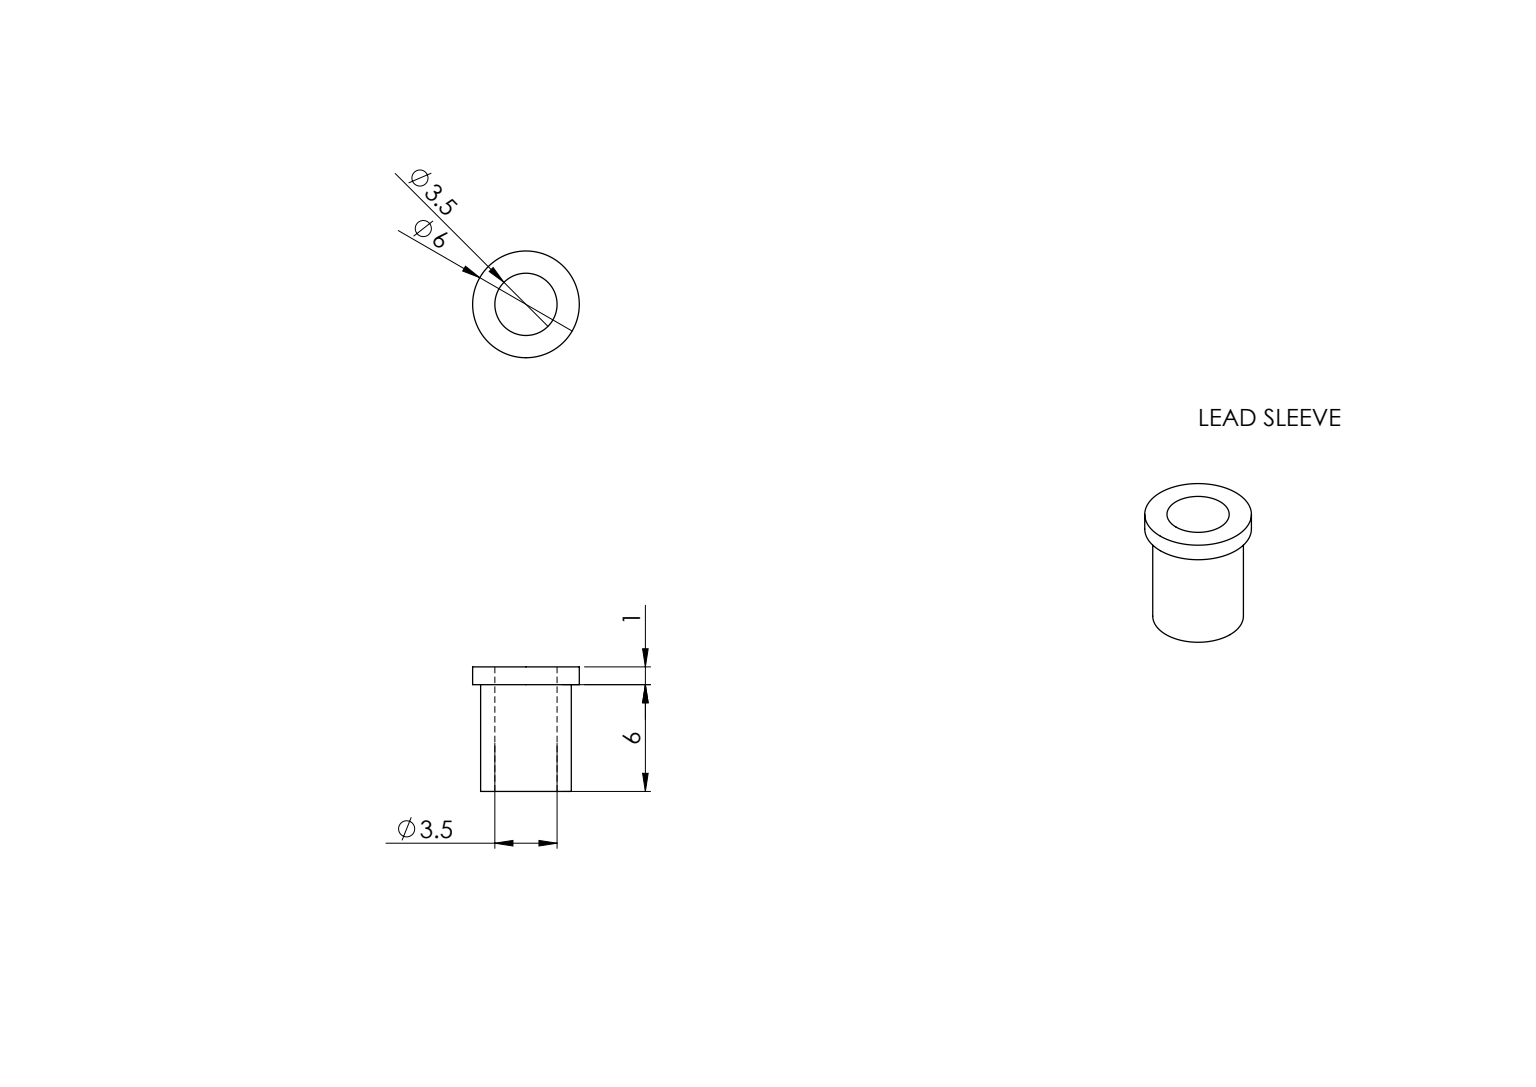
ISO-10303-21;
HEADER;
FILE_DESCRIPTION (('STEP AP214'),
    '1' );
FILE_NAME ('lead sleeve.step',
    '2026-10-27T10:49:47',
    ( '' ),
    ( '' ),
    'SwSTEP 2.0',
    'SolidWorks 2026',
    '' );
FILE_SCHEMA (( 'AUTOMOTIVE_DESIGN' ));
ENDSEC;

DATA;
#24=CARTESIAN_POINT ( 'NONE',  ( 0.000000000000000000, -53.00000000000000000, 0.000000000000000000 ) ) ;
#28=PRODUCT_DEFINITION_SHAPE ( 'NONE', 'NONE',  #6653 ) ;
#101=DIRECTION ( 'NONE',  ( 0.000000000000000000, 1.000000000000000000, 0.000000000000000000 ) ) ;
#135=ORIENTED_EDGE ( 'NONE', *, *, #4743, .T. ) ;
#208=ORIENTED_EDGE ( 'NONE', *, *, #3669, .T. ) ;
#212=EDGE_LOOP ( 'NONE', ( #4167, #4581 ) ) ;
#286=DIRECTION ( 'NONE',  ( -0.000000000000000000, 1.000000000000000000, -0.000000000000000000 ) ) ;
#296=VERTEX_POINT ( 'NONE', #8506 ) ;
#306=PRODUCT_DEFINITION_CONTEXT ( 'detailed design', #4038, 'design' ) ;
#328=CARTESIAN_POINT ( 'NONE',  ( 0.000000000000000000, -47.00000000000000000, 0.000000000000000000 ) ) ;
#391=EDGE_CURVE ( 'NONE', #8882, #738, #2591, .T. ) ;
#423=ORIENTED_EDGE ( 'NONE', *, *, #8631, .F. ) ;
#456=( NAMED_UNIT ( * ) SI_UNIT ( $, .STERADIAN. ) SOLID_ANGLE_UNIT ( ) );
#464=DIRECTION ( 'NONE',  ( -0.000000000000000000, -1.000000000000000000, -0.000000000000000000 ) ) ;
#468=ORIENTED_EDGE ( 'NONE', *, *, #7764, .T. ) ;
#469=CARTESIAN_POINT ( 'NONE',  ( 2.143131898507868051E-16, -53.00000000000000000, -1.749999999999999778 ) ) ;
#515=FACE_OUTER_BOUND ( 'NONE', #8742, .T. ) ;
#552=LINE ( 'NONE', #1253, #8953 ) ;
#596=CARTESIAN_POINT ( 'NONE',  ( 0.000000000000000000, -53.00000000000000000, 0.000000000000000000 ) ) ;
#631=ORIENTED_EDGE ( 'NONE', *, *, #8631, .T. ) ;
#673=ORIENTED_EDGE ( 'NONE', *, *, #5568, .T. ) ;
#711=CYLINDRICAL_SURFACE ( 'NONE', #5192, 1.749999999999999778 ) ;
#738=VERTEX_POINT ( 'NONE', #4144 ) ;
#791=VERTEX_POINT ( 'NONE', #4553 ) ;
#888=AXIS2_PLACEMENT_3D ( 'NONE', #4026, #9081, #6861 ) ;
#903=DIRECTION ( 'NONE',  ( 1.000000000000000000, 0.000000000000000000, 0.000000000000000000 ) ) ;
#945=AXIS2_PLACEMENT_3D ( 'NONE', #2361, #8822, #2458 ) ;
#968=ORIENTED_EDGE ( 'NONE', *, *, #8122, .T. ) ;
#1000=EDGE_CURVE ( 'NONE', #4607, #791, #3032, .T. ) ;
#1019=ORIENTED_EDGE ( 'NONE', *, *, #3908, .F. ) ;
#1038=VECTOR ( 'NONE', #2949, 1000.000000000000000 ) ;
#1070=CARTESIAN_POINT ( 'NONE',  ( 0.000000000000000000, -47.00000000000000000, 2.549999999999999822 ) ) ;
#1077=EDGE_CURVE ( 'NONE', #791, #6502, #552, .T. ) ;
#1085=DIRECTION ( 'NONE',  ( 0.000000000000000000, -1.000000000000000000, 0.000000000000000000 ) ) ;
#1134=CARTESIAN_POINT ( 'NONE',  ( 0.000000000000000000, -47.00000000000000000, 0.000000000000000000 ) ) ;
#1140=CARTESIAN_POINT ( 'NONE',  ( 0.000000000000000000, -47.00000000000000000, -2.999999999999999556 ) ) ;
#1143=LINE ( 'NONE', #6765, #5493 ) ;
#1210=SHAPE_DEFINITION_REPRESENTATION ( #28, #2490 ) ;
#1249=EDGE_CURVE ( 'NONE', #1724, #4568, #3611, .T. ) ;
#1253=CARTESIAN_POINT ( 'NONE',  ( 0.000000000000000000, -46.00000000000000000, -2.999999999999999556 ) ) ;
#1337=CARTESIAN_POINT ( 'NONE',  ( 0.000000000000000000, -53.00000000000000000, 0.000000000000000000 ) ) ;
#1386=ADVANCED_FACE ( 'NONE', ( #5610 ), #2170, .F. ) ;
#1441=DIRECTION ( 'NONE',  ( 0.000000000000000000, 0.000000000000000000, 1.000000000000000000 ) ) ;
#1472=DIRECTION ( 'NONE',  ( 0.000000000000000000, 1.000000000000000000, 0.000000000000000000 ) ) ;
#1490=DIRECTION ( 'NONE',  ( 0.000000000000000000, 1.000000000000000000, 0.000000000000000000 ) ) ;
#1516=UNCERTAINTY_MEASURE_WITH_UNIT (LENGTH_MEASURE( 1.000000000000000082E-05 ), #2714, 'distance_accuracy_value', 'NONE');
#1641=DIRECTION ( 'NONE',  ( 0.000000000000000000, 0.000000000000000000, 1.000000000000000000 ) ) ;
#1689=CARTESIAN_POINT ( 'NONE',  ( 0.000000000000000000, -53.00000000000000000, 2.549999999999999822 ) ) ;
#1724=VERTEX_POINT ( 'NONE', #8575 ) ;
#1835=CARTESIAN_POINT ( 'NONE',  ( 3.122849337825750419E-16, -53.00000000000000000, -2.549999999999999822 ) ) ;
#1844=VERTEX_POINT ( 'NONE', #469 ) ;
#1957=CARTESIAN_POINT ( 'NONE',  ( 0.000000000000000000, -53.00000000000000000, 0.000000000000000000 ) ) ;
#1993=DIRECTION ( 'NONE',  ( 0.000000000000000000, -1.000000000000000000, 0.000000000000000000 ) ) ;
#2043=DIRECTION ( 'NONE',  ( 0.000000000000000000, 0.000000000000000000, 1.000000000000000000 ) ) ;
#2148=MANIFOLD_SOLID_BREP ( 'Boss-Extrude1', #7133 ) ;
#2160=ORIENTED_EDGE ( 'NONE', *, *, #6275, .F. ) ;
#2170=CYLINDRICAL_SURFACE ( 'NONE', #2847, 1.749999999999999778 ) ;
#2214=DIRECTION ( 'NONE',  ( 1.000000000000000000, 0.000000000000000000, 0.000000000000000000 ) ) ;
#2216=AXIS2_PLACEMENT_3D ( 'NONE', #3437, #6390, #7094 ) ;
#2281=ORIENTED_EDGE ( 'NONE', *, *, #1000, .T. ) ;
#2361=CARTESIAN_POINT ( 'NONE',  ( 0.000000000000000000, -46.00000000000000000, 0.000000000000000000 ) ) ;
#2441=AXIS2_PLACEMENT_3D ( 'NONE', #5660, #7852, #2043 ) ;
#2458=DIRECTION ( 'NONE',  ( 0.000000000000000000, -0.000000000000000000, 1.000000000000000000 ) ) ;
#2464=DIRECTION ( 'NONE',  ( 0.000000000000000000, 0.000000000000000000, 1.000000000000000000 ) ) ;
#2479=FACE_BOUND ( 'NONE', #8500, .T. ) ;
#2490=SHAPE_REPRESENTATION ( 'lead sleeve', ( #888 ), #5908 ) ;
#2499=STYLED_ITEM ( 'NONE', ( #8555 ), #6298 ) ;
#2531=CARTESIAN_POINT ( 'NONE',  ( 0.000000000000000000, -53.00000000000000000, 0.000000000000000000 ) ) ;
#2560=DIRECTION ( 'NONE',  ( 0.000000000000000000, 1.000000000000000000, 0.000000000000000000 ) ) ;
#2583=DIRECTION ( 'NONE',  ( 0.000000000000000000, -1.000000000000000000, 0.000000000000000000 ) ) ;
#2591=CIRCLE ( 'NONE', #5546, 1.750000000000000222 ) ;
#2685=AXIS2_PLACEMENT_3D ( 'NONE', #8707, #101, #1641 ) ;
#2705=CARTESIAN_POINT ( 'NONE',  ( 0.000000000000000000, -46.00000000000000000, 0.000000000000000000 ) ) ;
#2714=( LENGTH_UNIT ( ) NAMED_UNIT ( * ) SI_UNIT ( .MILLI., .METRE. ) );
#2733=APPLICATION_CONTEXT ( 'automotive_design' ) ;
#2790=CARTESIAN_POINT ( 'NONE',  ( 0.000000000000000000, -53.00000000000000000, 0.000000000000000000 ) ) ;
#2804=( NAMED_UNIT ( * ) PLANE_ANGLE_UNIT ( ) SI_UNIT ( $, .RADIAN. ) );
#2806=ORIENTED_EDGE ( 'NONE', *, *, #8722, .T. ) ;
#2847=AXIS2_PLACEMENT_3D ( 'NONE', #596, #5567, #4991 ) ;
#2852=SURFACE_SIDE_STYLE ('',( #6497 ) ) ;
#2877=ADVANCED_FACE ( 'NONE', ( #7837 ), #711, .F. ) ;
#2921=LINE ( 'NONE', #5738, #5025 ) ;
#2949=DIRECTION ( 'NONE',  ( -0.000000000000000000, -1.000000000000000000, -0.000000000000000000 ) ) ;
#2991=ORIENTED_EDGE ( 'NONE', *, *, #5699, .F. ) ;
#3032=CIRCLE ( 'NONE', #7773, 2.999999999999999556 ) ;
#3139=AXIS2_PLACEMENT_3D ( 'NONE', #2790, #7100, #4360 ) ;
#3140=ORIENTED_EDGE ( 'NONE', *, *, #7764, .F. ) ;
#3143=FACE_OUTER_BOUND ( 'NONE', #5079, .T. ) ;
#3160=FACE_OUTER_BOUND ( 'NONE', #9177, .T. ) ;
#3183=ORIENTED_EDGE ( 'NONE', *, *, #8443, .F. ) ;
#3297=MECHANICAL_DESIGN_GEOMETRIC_PRESENTATION_REPRESENTATION('',(#8174),#4159);
#3303=FACE_OUTER_BOUND ( 'NONE', #6297, .T. ) ;
#3309=DIRECTION ( 'NONE',  ( 0.000000000000000000, 0.000000000000000000, 1.000000000000000000 ) ) ;
#3437=CARTESIAN_POINT ( 'NONE',  ( 0.000000000000000000, -46.00000000000000000, 0.000000000000000000 ) ) ;
#3447=CARTESIAN_POINT ( 'NONE',  ( 0.000000000000000000, -47.00000000000000000, 0.000000000000000000 ) ) ;
#3471=AXIS2_PLACEMENT_3D ( 'NONE', #1337, #7896, #2214 ) ;
#3502=LINE ( 'NONE', #7825, #9116 ) ;
#3515=DIRECTION ( 'NONE',  ( 0.000000000000000000, 0.000000000000000000, 1.000000000000000000 ) ) ;
#3538=( NAMED_UNIT ( * ) SI_UNIT ( $, .STERADIAN. ) SOLID_ANGLE_UNIT ( ) );
#3561=ORIENTED_EDGE ( 'NONE', *, *, #1000, .F. ) ;
#3611=CIRCLE ( 'NONE', #3471, 2.549999999999999822 ) ;
#3663=PLANE ( 'NONE',  #945 ) ;
#3669=EDGE_CURVE ( 'NONE', #6874, #296, #8611, .T. ) ;
#3767=AXIS2_PLACEMENT_3D ( 'NONE', #5405, #1490, #1441 ) ;
#3796=ADVANCED_FACE ( 'NONE', ( #7193 ), #4992, .T. ) ;
#3845=ORIENTED_EDGE ( 'NONE', *, *, #6275, .T. ) ;
#3896=ORIENTED_EDGE ( 'NONE', *, *, #1249, .F. ) ;
#3908=EDGE_CURVE ( 'NONE', #4607, #5775, #4385, .T. ) ;
#3986=DIRECTION ( 'NONE',  ( -0.000000000000000000, 1.000000000000000000, -0.000000000000000000 ) ) ;
#3997=( LENGTH_UNIT ( ) NAMED_UNIT ( * ) SI_UNIT ( .MILLI., .METRE. ) );
#4026=CARTESIAN_POINT ( 'NONE',  ( 0.000000000000000000, 0.000000000000000000, 0.000000000000000000 ) ) ;
#4038=APPLICATION_CONTEXT ( 'automotive_design' ) ;
#4048=CYLINDRICAL_SURFACE ( 'NONE', #6897, 2.549999999999999822 ) ;
#4111=CARTESIAN_POINT ( 'NONE',  ( 0.000000000000000000, -53.00000000000000000, 1.749999999999999778 ) ) ;
#4144=CARTESIAN_POINT ( 'NONE',  ( 2.143131898507868544E-16, -46.00000000000000000, -1.750000000000000222 ) ) ;
#4159=( GEOMETRIC_REPRESENTATION_CONTEXT ( 3 ) GLOBAL_UNCERTAINTY_ASSIGNED_CONTEXT ( ( #7422 ) ) GLOBAL_UNIT_ASSIGNED_CONTEXT ( ( #3997, #6778, #456 ) ) REPRESENTATION_CONTEXT ( 'NONE', 'WORKASPACE' ) );
#4167=ORIENTED_EDGE ( 'NONE', *, *, #391, .F. ) ;
#4175=FACE_OUTER_BOUND ( 'NONE', #8554, .T. ) ;
#4279=MECHANICAL_DESIGN_GEOMETRIC_PRESENTATION_REPRESENTATION('',(#2499),#6348);
#4360=DIRECTION ( 'NONE',  ( 0.000000000000000000, 0.000000000000000000, 1.000000000000000000 ) ) ;
#4385=LINE ( 'NONE', #7215, #1038 ) ;
#4400=ORIENTED_EDGE ( 'NONE', *, *, #5699, .T. ) ;
#4475=DIRECTION ( 'NONE',  ( 0.000000000000000000, -0.000000000000000000, 1.000000000000000000 ) ) ;
#4553=CARTESIAN_POINT ( 'NONE',  ( 0.000000000000000000, -46.00000000000000000, -2.999999999999999556 ) ) ;
#4568=VERTEX_POINT ( 'NONE', #1835 ) ;
#4581=ORIENTED_EDGE ( 'NONE', *, *, #6056, .F. ) ;
#4607=VERTEX_POINT ( 'NONE', #6052 ) ;
#4638=ORIENTED_EDGE ( 'NONE', *, *, #1077, .T. ) ;
#4643=CARTESIAN_POINT ( 'NONE',  ( 0.000000000000000000, -46.00000000000000000, 0.000000000000000000 ) ) ;
#4660=EDGE_LOOP ( 'NONE', ( #4753, #4816 ) ) ;
#4666=PLANE ( 'NONE',  #5776 ) ;
#4687=CARTESIAN_POINT ( 'NONE',  ( 0.000000000000000000, -53.00000000000000000, 0.000000000000000000 ) ) ;
#4690=CARTESIAN_POINT ( 'NONE',  ( 0.000000000000000000, -47.00000000000000000, 0.000000000000000000 ) ) ;
#4696=DIRECTION ( 'NONE',  ( 0.000000000000000000, 0.000000000000000000, -1.000000000000000000 ) ) ;
#4743=EDGE_CURVE ( 'NONE', #296, #6874, #7917, .T. ) ;
#4746=AXIS2_PLACEMENT_3D ( 'NONE', #4687, #6027, #8864 ) ;
#4750=ORIENTED_EDGE ( 'NONE', *, *, #4743, .F. ) ;
#4753=ORIENTED_EDGE ( 'NONE', *, *, #7099, .F. ) ;
#4783=CARTESIAN_POINT ( 'NONE',  ( 0.000000000000000000, -53.00000000000000000, 0.000000000000000000 ) ) ;
#4788=DIRECTION ( 'NONE',  ( 0.000000000000000000, 1.000000000000000000, 0.000000000000000000 ) ) ;
#4816=ORIENTED_EDGE ( 'NONE', *, *, #5422, .F. ) ;
#4825=DIRECTION ( 'NONE',  ( 1.000000000000000000, 0.000000000000000000, 0.000000000000000000 ) ) ;
#4906=EDGE_LOOP ( 'NONE', ( #468, #968, #8047, #3183 ) ) ;
#4921=PRODUCT ( 'lead sleeve', 'lead sleeve', '', ( #7531 ) ) ;
#4991=DIRECTION ( 'NONE',  ( 0.000000000000000000, 0.000000000000000000, 1.000000000000000000 ) ) ;
#4992=CYLINDRICAL_SURFACE ( 'NONE', #3139, 2.549999999999999822 ) ;
#4998=PRODUCT_DEFINITION_FORMATION_WITH_SPECIFIED_SOURCE ( 'ANY', '', #4921, .NOT_KNOWN. ) ;
#5025=VECTOR ( 'NONE', #7755, 1000.000000000000000 ) ;
#5079=EDGE_LOOP ( 'NONE', ( #5622, #3845 ) ) ;
#5160=ORIENTED_EDGE ( 'NONE', *, *, #8722, .F. ) ;
#5192=AXIS2_PLACEMENT_3D ( 'NONE', #7003, #8445, #3515 ) ;
#5303=EDGE_LOOP ( 'NONE', ( #2160, #673, #135, #5160 ) ) ;
#5355=DIRECTION ( 'NONE',  ( 0.000000000000000000, -0.000000000000000000, -1.000000000000000000 ) ) ;
#5384=VERTEX_POINT ( 'NONE', #4111 ) ;
#5405=CARTESIAN_POINT ( 'NONE',  ( 0.000000000000000000, -47.00000000000000000, 0.000000000000000000 ) ) ;
#5422=EDGE_CURVE ( 'NONE', #5775, #6502, #7482, .T. ) ;
#5429=DIRECTION ( 'NONE',  ( 0.000000000000000000, -1.000000000000000000, 0.000000000000000000 ) ) ;
#5470=ORIENTED_EDGE ( 'NONE', *, *, #8443, .T. ) ;
#5493=VECTOR ( 'NONE', #3986, 1000.000000000000000 ) ;
#5546=AXIS2_PLACEMENT_3D ( 'NONE', #7287, #1472, #6443 ) ;
#5553=AXIS2_PLACEMENT_3D ( 'NONE', #1957, #6929, #6183 ) ;
#5567=DIRECTION ( 'NONE',  ( -0.000000000000000000, 1.000000000000000000, -0.000000000000000000 ) ) ;
#5568=EDGE_CURVE ( 'NONE', #4568, #296, #3502, .T. ) ;
#5610=FACE_OUTER_BOUND ( 'NONE', #4906, .T. ) ;
#5622=ORIENTED_EDGE ( 'NONE', *, *, #1249, .T. ) ;
#5660=CARTESIAN_POINT ( 'NONE',  ( 0.000000000000000000, -46.00000000000000000, 0.000000000000000000 ) ) ;
#5669=SHAPE_REPRESENTATION_RELATIONSHIP ( 'NONE' , 'NONE' ,  #2490, #6298 ) ;
#5699=EDGE_CURVE ( 'NONE', #1844, #5384, #8960, .T. ) ;
#5704=ADVANCED_FACE ( 'NONE', ( #3303 ), #4048, .T. ) ;
#5712=SURFACE_STYLE_USAGE ( .BOTH. , #2852 ) ;
#5738=CARTESIAN_POINT ( 'NONE',  ( 2.143131898507868051E-16, -53.00000000000000000, -1.749999999999999778 ) ) ;
#5775=VERTEX_POINT ( 'NONE', #8964 ) ;
#5776=AXIS2_PLACEMENT_3D ( 'NONE', #2531, #1085, #5355 ) ;
#5807=CARTESIAN_POINT ( 'NONE',  ( 0.000000000000000000, -46.00000000000000000, 1.750000000000000222 ) ) ;
#5808=ORIENTED_EDGE ( 'NONE', *, *, #8122, .F. ) ;
#5864=PLANE ( 'NONE',  #6294 ) ;
#5872=ADVANCED_FACE ( 'NONE', ( #2479, #8104 ), #5864, .F. ) ;
#5908=( GEOMETRIC_REPRESENTATION_CONTEXT ( 3 ) GLOBAL_UNCERTAINTY_ASSIGNED_CONTEXT ( ( #1516 ) ) GLOBAL_UNIT_ASSIGNED_CONTEXT ( ( #2714, #6098, #6983 ) ) REPRESENTATION_CONTEXT ( 'NONE', 'WORKASPACE' ) );
#5980=FACE_BOUND ( 'NONE', #212, .T. ) ;
#5994=CIRCLE ( 'NONE', #7783, 2.549999999999999822 ) ;
#6024=ORIENTED_EDGE ( 'NONE', *, *, #391, .T. ) ;
#6027=DIRECTION ( 'NONE',  ( 0.000000000000000000, -1.000000000000000000, 0.000000000000000000 ) ) ;
#6052=CARTESIAN_POINT ( 'NONE',  ( 3.673940397442059375E-16, -46.00000000000000000, 2.999999999999999556 ) ) ;
#6056=EDGE_CURVE ( 'NONE', #738, #8882, #6431, .T. ) ;
#6076=DIRECTION ( 'NONE',  ( -0.000000000000000000, -1.000000000000000000, -0.000000000000000000 ) ) ;
#6098=( NAMED_UNIT ( * ) PLANE_ANGLE_UNIT ( ) SI_UNIT ( $, .RADIAN. ) );
#6119=ORIENTED_EDGE ( 'NONE', *, *, #5422, .T. ) ;
#6139=CYLINDRICAL_SURFACE ( 'NONE', #6819, 2.999999999999999556 ) ;
#6174=ADVANCED_FACE ( 'NONE', ( #3160, #5980 ), #3663, .T. ) ;
#6183=DIRECTION ( 'NONE',  ( 0.000000000000000000, 0.000000000000000000, -1.000000000000000000 ) ) ;
#6275=EDGE_CURVE ( 'NONE', #4568, #1724, #5994, .T. ) ;
#6294=AXIS2_PLACEMENT_3D ( 'NONE', #328, #8704, #4475 ) ;
#6297=EDGE_LOOP ( 'NONE', ( #6732, #3896, #2806, #208 ) ) ;
#6298=ADVANCED_BREP_SHAPE_REPRESENTATION ( '', ( #2148, #888 ), #5908 ) ;
#6348=( GEOMETRIC_REPRESENTATION_CONTEXT ( 3 ) GLOBAL_UNCERTAINTY_ASSIGNED_CONTEXT ( ( #6534 ) ) GLOBAL_UNIT_ASSIGNED_CONTEXT ( ( #7068, #2804, #3538 ) ) REPRESENTATION_CONTEXT ( 'NONE', 'WORKASPACE' ) );
#6390=DIRECTION ( 'NONE',  ( -0.000000000000000000, -1.000000000000000000, -0.000000000000000000 ) ) ;
#6431=CIRCLE ( 'NONE', #2441, 1.750000000000000222 ) ;
#6443=DIRECTION ( 'NONE',  ( 0.000000000000000000, 0.000000000000000000, 1.000000000000000000 ) ) ;
#6497=SURFACE_STYLE_FILL_AREA ( #7728 ) ;
#6502=VERTEX_POINT ( 'NONE', #1140 ) ;
#6534=UNCERTAINTY_MEASURE_WITH_UNIT (LENGTH_MEASURE( 1.000000000000000082E-05 ), #7068, 'distance_accuracy_value', 'NONE');
#6653=PRODUCT_DEFINITION ( 'UNKNOWN', '', #4998, #306 ) ;
#6732=ORIENTED_EDGE ( 'NONE', *, *, #5568, .F. ) ;
#6765=CARTESIAN_POINT ( 'NONE',  ( 0.000000000000000000, -53.00000000000000000, 1.749999999999999778 ) ) ;
#6778=( NAMED_UNIT ( * ) PLANE_ANGLE_UNIT ( ) SI_UNIT ( $, .RADIAN. ) );
#6819=AXIS2_PLACEMENT_3D ( 'NONE', #2705, #464, #4696 ) ;
#6861=DIRECTION ( 'NONE',  ( 1.000000000000000000, 0.000000000000000000, 0.000000000000000000 ) ) ;
#6874=VERTEX_POINT ( 'NONE', #1070 ) ;
#6897=AXIS2_PLACEMENT_3D ( 'NONE', #4783, #8186, #2464 ) ;
#6929=DIRECTION ( 'NONE',  ( 0.000000000000000000, -1.000000000000000000, 0.000000000000000000 ) ) ;
#6983=( NAMED_UNIT ( * ) SI_UNIT ( $, .STERADIAN. ) SOLID_ANGLE_UNIT ( ) );
#7003=CARTESIAN_POINT ( 'NONE',  ( 0.000000000000000000, -53.00000000000000000, 0.000000000000000000 ) ) ;
#7068=( LENGTH_UNIT ( ) NAMED_UNIT ( * ) SI_UNIT ( .MILLI., .METRE. ) );
#7094=DIRECTION ( 'NONE',  ( 0.000000000000000000, 0.000000000000000000, -1.000000000000000000 ) ) ;
#7096=ADVANCED_FACE ( 'NONE', ( #515 ), #6139, .T. ) ;
#7099=EDGE_CURVE ( 'NONE', #6502, #5775, #7566, .T. ) ;
#7100=DIRECTION ( 'NONE',  ( -0.000000000000000000, 1.000000000000000000, -0.000000000000000000 ) ) ;
#7115=CIRCLE ( 'NONE', #4746, 1.749999999999999778 ) ;
#7133=CLOSED_SHELL ( 'NONE', ( #7096, #1386, #3796, #8797, #5704, #2877, #6174, #5872, #7979 ) ) ;
#7161=EDGE_LOOP ( 'NONE', ( #3140, #2991 ) ) ;
#7193=FACE_OUTER_BOUND ( 'NONE', #5303, .T. ) ;
#7215=CARTESIAN_POINT ( 'NONE',  ( 3.673940397442059375E-16, -46.00000000000000000, 2.999999999999999556 ) ) ;
#7282=AXIS2_PLACEMENT_3D ( 'NONE', #4690, #5429, #4825 ) ;
#7287=CARTESIAN_POINT ( 'NONE',  ( 0.000000000000000000, -46.00000000000000000, 0.000000000000000000 ) ) ;
#7299=ORIENTED_EDGE ( 'NONE', *, *, #7099, .T. ) ;
#7392=COLOUR_RGB ( '',0.8941176470588234615, 0.8941176470588234615, 0.8941176470588234615 ) ;
#7422=UNCERTAINTY_MEASURE_WITH_UNIT (LENGTH_MEASURE( 1.000000000000000082E-05 ), #3997, 'distance_accuracy_value', 'NONE');
#7482=CIRCLE ( 'NONE', #3767, 2.999999999999999556 ) ;
#7484=DIRECTION ( 'NONE',  ( 0.000000000000000000, 0.000000000000000000, 1.000000000000000000 ) ) ;
#7530=ORIENTED_EDGE ( 'NONE', *, *, #3908, .T. ) ;
#7531=PRODUCT_CONTEXT ( 'NONE', #2733, 'mechanical' ) ;
#7544=ORIENTED_EDGE ( 'NONE', *, *, #3669, .F. ) ;
#7566=CIRCLE ( 'NONE', #8747, 2.999999999999999556 ) ;
#7728=FILL_AREA_STYLE ('',( #8473 ) ) ;
#7755=DIRECTION ( 'NONE',  ( -0.000000000000000000, 1.000000000000000000, -0.000000000000000000 ) ) ;
#7764=EDGE_CURVE ( 'NONE', #5384, #1844, #7115, .T. ) ;
#7773=AXIS2_PLACEMENT_3D ( 'NONE', #4643, #2560, #7484 ) ;
#7780=DIRECTION ( 'NONE',  ( -0.000000000000000000, 1.000000000000000000, -0.000000000000000000 ) ) ;
#7783=AXIS2_PLACEMENT_3D ( 'NONE', #24, #1993, #903 ) ;
#7825=CARTESIAN_POINT ( 'NONE',  ( 3.122849337825750419E-16, -53.00000000000000000, -2.549999999999999822 ) ) ;
#7837=FACE_OUTER_BOUND ( 'NONE', #8770, .T. ) ;
#7852=DIRECTION ( 'NONE',  ( 0.000000000000000000, 1.000000000000000000, 0.000000000000000000 ) ) ;
#7892=CYLINDRICAL_SURFACE ( 'NONE', #2216, 2.999999999999999556 ) ;
#7896=DIRECTION ( 'NONE',  ( 0.000000000000000000, -1.000000000000000000, 0.000000000000000000 ) ) ;
#7917=CIRCLE ( 'NONE', #8064, 2.549999999999999822 ) ;
#7921=LINE ( 'NONE', #1689, #8761 ) ;
#7979=ADVANCED_FACE ( 'NONE', ( #4175 ), #7892, .T. ) ;
#8047=ORIENTED_EDGE ( 'NONE', *, *, #6056, .T. ) ;
#8064=AXIS2_PLACEMENT_3D ( 'NONE', #1134, #2583, #8847 ) ;
#8104=FACE_OUTER_BOUND ( 'NONE', #4660, .T. ) ;
#8108=FACE_BOUND ( 'NONE', #7161, .T. ) ;
#8122=EDGE_CURVE ( 'NONE', #1844, #738, #2921, .T. ) ;
#8174=STYLED_ITEM('',(#9239),#2148);
#8186=DIRECTION ( 'NONE',  ( -0.000000000000000000, 1.000000000000000000, -0.000000000000000000 ) ) ;
#8323=CIRCLE ( 'NONE', #2685, 2.999999999999999556 ) ;
#8443=EDGE_CURVE ( 'NONE', #5384, #8882, #1143, .T. ) ;
#8445=DIRECTION ( 'NONE',  ( -0.000000000000000000, 1.000000000000000000, -0.000000000000000000 ) ) ;
#8473=FILL_AREA_STYLE_COLOUR ( '', #7392 ) ;
#8500=EDGE_LOOP ( 'NONE', ( #7544, #4750 ) ) ;
#8506=CARTESIAN_POINT ( 'NONE',  ( 3.122849337825750419E-16, -47.00000000000000000, -2.549999999999999822 ) ) ;
#8554=EDGE_LOOP ( 'NONE', ( #1019, #423, #4638, #7299 ) ) ;
#8555=PRESENTATION_STYLE_ASSIGNMENT (( #5712 ) ) ;
#8575=CARTESIAN_POINT ( 'NONE',  ( 0.000000000000000000, -53.00000000000000000, 2.549999999999999822 ) ) ;
#8611=CIRCLE ( 'NONE', #7282, 2.549999999999999822 ) ;
#8631=EDGE_CURVE ( 'NONE', #791, #4607, #8323, .T. ) ;
#8704=DIRECTION ( 'NONE',  ( 0.000000000000000000, 1.000000000000000000, 0.000000000000000000 ) ) ;
#8707=CARTESIAN_POINT ( 'NONE',  ( 0.000000000000000000, -46.00000000000000000, 0.000000000000000000 ) ) ;
#8722=EDGE_CURVE ( 'NONE', #1724, #6874, #7921, .T. ) ;
#8742=EDGE_LOOP ( 'NONE', ( #3561, #7530, #6119, #8821 ) ) ;
#8747=AXIS2_PLACEMENT_3D ( 'NONE', #3447, #4788, #3309 ) ;
#8761=VECTOR ( 'NONE', #286, 1000.000000000000000 ) ;
#8770=EDGE_LOOP ( 'NONE', ( #5808, #4400, #5470, #6024 ) ) ;
#8797=ADVANCED_FACE ( 'NONE', ( #3143, #8108 ), #4666, .T. ) ;
#8821=ORIENTED_EDGE ( 'NONE', *, *, #1077, .F. ) ;
#8822=DIRECTION ( 'NONE',  ( 0.000000000000000000, 1.000000000000000000, 0.000000000000000000 ) ) ;
#8847=DIRECTION ( 'NONE',  ( 1.000000000000000000, 0.000000000000000000, 0.000000000000000000 ) ) ;
#8864=DIRECTION ( 'NONE',  ( 0.000000000000000000, 0.000000000000000000, -1.000000000000000000 ) ) ;
#8882=VERTEX_POINT ( 'NONE', #5807 ) ;
#8953=VECTOR ( 'NONE', #6076, 1000.000000000000000 ) ;
#8960=CIRCLE ( 'NONE', #5553, 1.749999999999999778 ) ;
#8964=CARTESIAN_POINT ( 'NONE',  ( 3.673940397442059375E-16, -47.00000000000000000, 2.999999999999999556 ) ) ;
#9081=DIRECTION ( 'NONE',  ( 0.000000000000000000, 0.000000000000000000, 1.000000000000000000 ) ) ;
#9116=VECTOR ( 'NONE', #7780, 1000.000000000000000 ) ;
#9177=EDGE_LOOP ( 'NONE', ( #631, #2281 ) ) ;
#9233=COLOUR_RGB('Off White',0.89,0.88,0.83);
#9234=FILL_AREA_STYLE_COLOUR('',#9233);
#9235=FILL_AREA_STYLE('',(#9234));
#9236=SURFACE_STYLE_FILL_AREA(#9235);
#9237=SURFACE_SIDE_STYLE('',(#9236));
#9238=SURFACE_STYLE_USAGE(.BOTH.,#9237);
#9239=PRESENTATION_STYLE_ASSIGNMENT((#9238));
ENDSEC;
END-ISO-10303-21;
